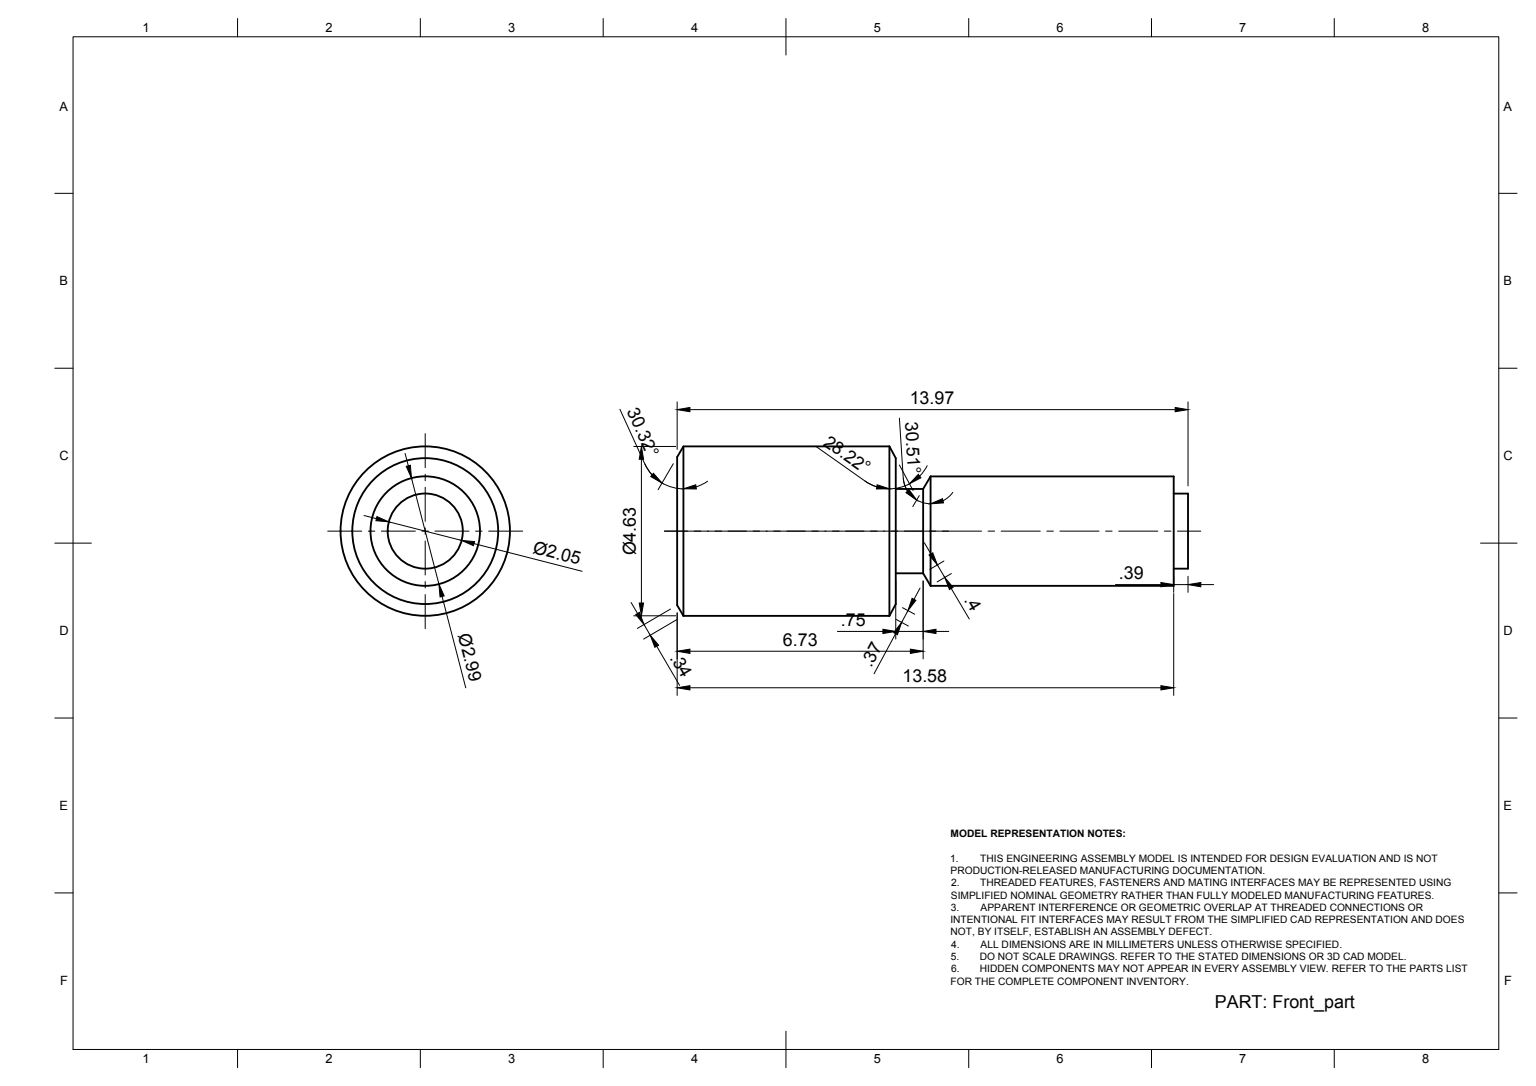
ISO-10303-21;
HEADER;
/* Generated by software containing ST-Developer
 * from STEP Tools, Inc. (www.steptools.com) 
 */

FILE_DESCRIPTION(
/* description */ (''),
/* implementation_level */ '2;1');

FILE_NAME(
/* name */ 'Front_part.step',
/* time_stamp */ '2026-10-05T00:51:14-07:00',
/* author */ (''),
/* organization */ (''),
/* preprocessor_version */ 'ST-DEVELOPER v20.2',
/* originating_system */ 'Autodesk Translation Framework v15.15.0.0',
/* authorisation */ '');

FILE_SCHEMA (('AUTOMOTIVE_DESIGN { 1 0 10303 214 3 1 1 }'));
ENDSEC;

DATA;
#10=MECHANICAL_DESIGN_GEOMETRIC_PRESENTATION_REPRESENTATION('',(#390),#4613);
#55=CONICAL_SURFACE('',#1766,1.32430878211522,1.03823317791294);
#56=CONICAL_SURFACE('',#1773,2.15547938178353,1.07831899445638);
#57=CONICAL_SURFACE('',#1777,2.17072351166958,1.04154954596305);
#77=FACE_BOUND('',#558,.T.);
#78=FACE_BOUND('',#563,.T.);
#79=FACE_BOUND('',#569,.T.);
#105=PLANE('',#1771);
#106=PLANE('',#1779);
#107=PLANE('',#1783);
#108=PLANE('',#1784);
#109=PLANE('',#1788);
#191=LINE('',#2638,#274);
#192=LINE('',#2643,#275);
#193=LINE('',#2650,#276);
#194=LINE('',#2654,#277);
#195=LINE('',#2657,#278);
#196=LINE('',#2665,#279);
#197=LINE('',#2673,#280);
#198=LINE('',#2678,#281);
#274=VECTOR('',#2082,1.32430878211522);
#275=VECTOR('',#2089,1.15283995859749);
#276=VECTOR('',#2098,2.15547938178353);
#277=VECTOR('',#2103,2.3164003912567);
#278=VECTOR('',#2106,2.17072351166958);
#279=VECTOR('',#2117,0.94209020647254);
#280=VECTOR('',#2128,1.02706997925809);
#281=VECTOR('',#2135,1.49577760563294);
#345=CYLINDRICAL_SURFACE('',#1769,1.15283995859749);
#346=CYLINDRICAL_SURFACE('',#1775,2.3164003912567);
#347=CYLINDRICAL_SURFACE('',#1781,0.94209020647254);
#348=CYLINDRICAL_SURFACE('',#1786,1.02706997925809);
#349=CYLINDRICAL_SURFACE('',#1790,1.49577760563294);
#374=SHAPE_REPRESENTATION_RELATIONSHIP('SRR','None',#4648,#382);
#382=ADVANCED_BREP_SHAPE_REPRESENTATION('',(#398),#4608);
#390=STYLED_ITEM('',(#4695),#398);
#398=MANIFOLD_SOLID_BREP('Body1',#1597);
#439=FACE_OUTER_BOUND('',#555,.T.);
#440=FACE_OUTER_BOUND('',#556,.T.);
#441=FACE_OUTER_BOUND('',#557,.T.);
#442=FACE_OUTER_BOUND('',#559,.T.);
#443=FACE_OUTER_BOUND('',#560,.T.);
#444=FACE_OUTER_BOUND('',#561,.T.);
#445=FACE_OUTER_BOUND('',#562,.T.);
#446=FACE_OUTER_BOUND('',#564,.T.);
#447=FACE_OUTER_BOUND('',#565,.T.);
#448=FACE_OUTER_BOUND('',#566,.T.);
#449=FACE_OUTER_BOUND('',#567,.T.);
#450=FACE_OUTER_BOUND('',#568,.T.);
#451=FACE_OUTER_BOUND('',#570,.T.);
#555=EDGE_LOOP('',(#1205,#1206,#1207,#1208));
#556=EDGE_LOOP('',(#1209,#1210,#1211,#1212));
#557=EDGE_LOOP('',(#1213));
#558=EDGE_LOOP('',(#1214));
#559=EDGE_LOOP('',(#1215,#1216,#1217,#1218));
#560=EDGE_LOOP('',(#1219,#1220,#1221,#1222));
#561=EDGE_LOOP('',(#1223,#1224,#1225,#1226));
#562=EDGE_LOOP('',(#1227));
#563=EDGE_LOOP('',(#1228));
#564=EDGE_LOOP('',(#1229,#1230,#1231,#1232));
#565=EDGE_LOOP('',(#1233));
#566=EDGE_LOOP('',(#1234));
#567=EDGE_LOOP('',(#1235,#1236,#1237,#1238));
#568=EDGE_LOOP('',(#1239));
#569=EDGE_LOOP('',(#1240));
#570=EDGE_LOOP('',(#1241,#1242,#1243,#1244));
#673=CIRCLE('',#1767,1.49577760563294);
#674=CIRCLE('',#1768,1.15283995859749);
#675=CIRCLE('',#1770,1.15283995859749);
#676=CIRCLE('',#1772,1.99455837231036);
#677=CIRCLE('',#1774,2.3164003912567);
#678=CIRCLE('',#1776,2.3164003912567);
#679=CIRCLE('',#1778,2.02504663208246);
#680=CIRCLE('',#1780,0.94209020647254);
#681=CIRCLE('',#1782,0.94209020647254);
#682=CIRCLE('',#1785,1.02706997925809);
#683=CIRCLE('',#1787,1.02706997925809);
#684=CIRCLE('',#1789,1.49577760563294);
#774=VERTEX_POINT('',#2635);
#775=VERTEX_POINT('',#2637);
#776=VERTEX_POINT('',#2641);
#777=VERTEX_POINT('',#2645);
#778=VERTEX_POINT('',#2648);
#779=VERTEX_POINT('',#2652);
#780=VERTEX_POINT('',#2656);
#781=VERTEX_POINT('',#2660);
#782=VERTEX_POINT('',#2663);
#783=VERTEX_POINT('',#2668);
#784=VERTEX_POINT('',#2671);
#785=VERTEX_POINT('',#2675);
#930=EDGE_CURVE('',#774,#774,#673,.T.);
#931=EDGE_CURVE('',#774,#775,#191,.T.);
#932=EDGE_CURVE('',#775,#775,#674,.T.);
#933=EDGE_CURVE('',#776,#776,#675,.T.);
#934=EDGE_CURVE('',#776,#775,#192,.T.);
#935=EDGE_CURVE('',#777,#777,#676,.T.);
#936=EDGE_CURVE('',#778,#778,#677,.T.);
#937=EDGE_CURVE('',#778,#777,#193,.T.);
#938=EDGE_CURVE('',#779,#779,#678,.T.);
#939=EDGE_CURVE('',#779,#778,#194,.T.);
#940=EDGE_CURVE('',#779,#780,#195,.T.);
#941=EDGE_CURVE('',#780,#780,#679,.T.);
#942=EDGE_CURVE('',#781,#781,#680,.T.);
#943=EDGE_CURVE('',#782,#782,#681,.T.);
#944=EDGE_CURVE('',#782,#781,#196,.T.);
#945=EDGE_CURVE('',#783,#783,#682,.T.);
#946=EDGE_CURVE('',#784,#784,#683,.T.);
#947=EDGE_CURVE('',#784,#783,#197,.T.);
#948=EDGE_CURVE('',#785,#785,#684,.T.);
#949=EDGE_CURVE('',#774,#785,#198,.T.);
#1205=ORIENTED_EDGE('',*,*,#930,.T.);
#1206=ORIENTED_EDGE('',*,*,#931,.T.);
#1207=ORIENTED_EDGE('',*,*,#932,.F.);
#1208=ORIENTED_EDGE('',*,*,#931,.F.);
#1209=ORIENTED_EDGE('',*,*,#933,.F.);
#1210=ORIENTED_EDGE('',*,*,#934,.T.);
#1211=ORIENTED_EDGE('',*,*,#932,.T.);
#1212=ORIENTED_EDGE('',*,*,#934,.F.);
#1213=ORIENTED_EDGE('',*,*,#935,.F.);
#1214=ORIENTED_EDGE('',*,*,#933,.T.);
#1215=ORIENTED_EDGE('',*,*,#936,.F.);
#1216=ORIENTED_EDGE('',*,*,#937,.T.);
#1217=ORIENTED_EDGE('',*,*,#935,.T.);
#1218=ORIENTED_EDGE('',*,*,#937,.F.);
#1219=ORIENTED_EDGE('',*,*,#938,.F.);
#1220=ORIENTED_EDGE('',*,*,#939,.T.);
#1221=ORIENTED_EDGE('',*,*,#936,.T.);
#1222=ORIENTED_EDGE('',*,*,#939,.F.);
#1223=ORIENTED_EDGE('',*,*,#938,.T.);
#1224=ORIENTED_EDGE('',*,*,#940,.T.);
#1225=ORIENTED_EDGE('',*,*,#941,.F.);
#1226=ORIENTED_EDGE('',*,*,#940,.F.);
#1227=ORIENTED_EDGE('',*,*,#941,.T.);
#1228=ORIENTED_EDGE('',*,*,#942,.F.);
#1229=ORIENTED_EDGE('',*,*,#943,.F.);
#1230=ORIENTED_EDGE('',*,*,#944,.T.);
#1231=ORIENTED_EDGE('',*,*,#942,.T.);
#1232=ORIENTED_EDGE('',*,*,#944,.F.);
#1233=ORIENTED_EDGE('',*,*,#943,.T.);
#1234=ORIENTED_EDGE('',*,*,#945,.F.);
#1235=ORIENTED_EDGE('',*,*,#946,.F.);
#1236=ORIENTED_EDGE('',*,*,#947,.T.);
#1237=ORIENTED_EDGE('',*,*,#945,.T.);
#1238=ORIENTED_EDGE('',*,*,#947,.F.);
#1239=ORIENTED_EDGE('',*,*,#948,.F.);
#1240=ORIENTED_EDGE('',*,*,#946,.T.);
#1241=ORIENTED_EDGE('',*,*,#930,.F.);
#1242=ORIENTED_EDGE('',*,*,#949,.T.);
#1243=ORIENTED_EDGE('',*,*,#948,.T.);
#1244=ORIENTED_EDGE('',*,*,#949,.F.);
#1524=ADVANCED_FACE('',(#439),#55,.T.);
#1525=ADVANCED_FACE('',(#440),#345,.T.);
#1526=ADVANCED_FACE('',(#441,#77),#105,.T.);
#1527=ADVANCED_FACE('',(#442),#56,.T.);
#1528=ADVANCED_FACE('',(#443),#346,.T.);
#1529=ADVANCED_FACE('',(#444),#57,.T.);
#1530=ADVANCED_FACE('',(#445,#78),#106,.T.);
#1531=ADVANCED_FACE('',(#446),#347,.F.);
#1532=ADVANCED_FACE('',(#447),#107,.T.);
#1533=ADVANCED_FACE('',(#448),#108,.T.);
#1534=ADVANCED_FACE('',(#449),#348,.T.);
#1535=ADVANCED_FACE('',(#450,#79),#109,.T.);
#1536=ADVANCED_FACE('',(#451),#349,.T.);
#1597=CLOSED_SHELL('',(#1524,#1525,#1526,#1527,#1528,#1529,#1530,#1531,
#1532,#1533,#1534,#1535,#1536));
#1765=AXIS2_PLACEMENT_3D('',#2633,#2076,#2077);
#1766=AXIS2_PLACEMENT_3D('',#2634,#2078,#2079);
#1767=AXIS2_PLACEMENT_3D('',#2636,#2080,#2081);
#1768=AXIS2_PLACEMENT_3D('',#2639,#2083,#2084);
#1769=AXIS2_PLACEMENT_3D('',#2640,#2085,#2086);
#1770=AXIS2_PLACEMENT_3D('',#2642,#2087,#2088);
#1771=AXIS2_PLACEMENT_3D('',#2644,#2090,#2091);
#1772=AXIS2_PLACEMENT_3D('',#2646,#2092,#2093);
#1773=AXIS2_PLACEMENT_3D('',#2647,#2094,#2095);
#1774=AXIS2_PLACEMENT_3D('',#2649,#2096,#2097);
#1775=AXIS2_PLACEMENT_3D('',#2651,#2099,#2100);
#1776=AXIS2_PLACEMENT_3D('',#2653,#2101,#2102);
#1777=AXIS2_PLACEMENT_3D('',#2655,#2104,#2105);
#1778=AXIS2_PLACEMENT_3D('',#2658,#2107,#2108);
#1779=AXIS2_PLACEMENT_3D('',#2659,#2109,#2110);
#1780=AXIS2_PLACEMENT_3D('',#2661,#2111,#2112);
#1781=AXIS2_PLACEMENT_3D('',#2662,#2113,#2114);
#1782=AXIS2_PLACEMENT_3D('',#2664,#2115,#2116);
#1783=AXIS2_PLACEMENT_3D('',#2666,#2118,#2119);
#1784=AXIS2_PLACEMENT_3D('',#2667,#2120,#2121);
#1785=AXIS2_PLACEMENT_3D('',#2669,#2122,#2123);
#1786=AXIS2_PLACEMENT_3D('',#2670,#2124,#2125);
#1787=AXIS2_PLACEMENT_3D('',#2672,#2126,#2127);
#1788=AXIS2_PLACEMENT_3D('',#2674,#2129,#2130);
#1789=AXIS2_PLACEMENT_3D('',#2676,#2131,#2132);
#1790=AXIS2_PLACEMENT_3D('',#2677,#2133,#2134);
#2076=DIRECTION('axis',(0.,0.,1.));
#2077=DIRECTION('refdir',(1.,0.,0.));
#2078=DIRECTION('center_axis',(-1.,0.,0.));
#2079=DIRECTION('ref_axis',(0.,0.,-1.));
#2080=DIRECTION('center_axis',(1.,0.,0.));
#2081=DIRECTION('ref_axis',(0.,0.,-1.));
#2082=DIRECTION('',(0.507743181153061,-1.05504360309624E-16,-0.861508480511115));
#2083=DIRECTION('center_axis',(1.,0.,0.));
#2084=DIRECTION('ref_axis',(0.,0.,-1.));
#2085=DIRECTION('center_axis',(1.,0.,0.));
#2086=DIRECTION('ref_axis',(0.,0.,-1.));
#2087=DIRECTION('center_axis',(1.,0.,0.));
#2088=DIRECTION('ref_axis',(0.,0.,-1.));
#2089=DIRECTION('',(-1.,0.,0.));
#2090=DIRECTION('center_axis',(-1.,0.,0.));
#2091=DIRECTION('ref_axis',(0.,0.,1.));
#2092=DIRECTION('center_axis',(1.,0.,0.));
#2093=DIRECTION('ref_axis',(0.,0.,-1.));
#2094=DIRECTION('center_axis',(1.,0.,0.));
#2095=DIRECTION('ref_axis',(0.,0.,-1.));
#2096=DIRECTION('center_axis',(1.,0.,0.));
#2097=DIRECTION('ref_axis',(0.,0.,-1.));
#2098=DIRECTION('',(-0.472810273503224,1.07911498508989E-16,-0.88116425555614));
#2099=DIRECTION('center_axis',(1.,0.,0.));
#2100=DIRECTION('ref_axis',(0.,0.,-1.));
#2101=DIRECTION('center_axis',(1.,0.,0.));
#2102=DIRECTION('ref_axis',(0.,0.,-1.));
#2103=DIRECTION('',(-1.,0.,0.));
#2104=DIRECTION('center_axis',(-1.,0.,0.));
#2105=DIRECTION('ref_axis',(0.,0.,-1.));
#2106=DIRECTION('',(0.504883315037955,-1.0570999352361E-16,-0.863187603129404));
#2107=DIRECTION('center_axis',(1.,0.,0.));
#2108=DIRECTION('ref_axis',(0.,0.,-1.));
#2109=DIRECTION('center_axis',(1.,0.,0.));
#2110=DIRECTION('ref_axis',(0.,0.,-1.));
#2111=DIRECTION('center_axis',(1.,0.,0.));
#2112=DIRECTION('ref_axis',(0.,0.,-1.));
#2113=DIRECTION('center_axis',(1.,0.,0.));
#2114=DIRECTION('ref_axis',(0.,0.,-1.));
#2115=DIRECTION('center_axis',(1.,0.,0.));
#2116=DIRECTION('ref_axis',(0.,0.,-1.));
#2117=DIRECTION('',(1.,0.,0.));
#2118=DIRECTION('center_axis',(1.,0.,0.));
#2119=DIRECTION('ref_axis',(0.,0.,-1.));
#2120=DIRECTION('center_axis',(-1.,0.,0.));
#2121=DIRECTION('ref_axis',(0.,0.,1.));
#2122=DIRECTION('center_axis',(1.,0.,0.));
#2123=DIRECTION('ref_axis',(0.,0.,-1.));
#2124=DIRECTION('center_axis',(1.,0.,0.));
#2125=DIRECTION('ref_axis',(0.,0.,-1.));
#2126=DIRECTION('center_axis',(1.,0.,0.));
#2127=DIRECTION('ref_axis',(0.,0.,-1.));
#2128=DIRECTION('',(-1.,0.,0.));
#2129=DIRECTION('center_axis',(-1.,0.,0.));
#2130=DIRECTION('ref_axis',(0.,0.,1.));
#2131=DIRECTION('center_axis',(1.,0.,0.));
#2132=DIRECTION('ref_axis',(0.,0.,-1.));
#2133=DIRECTION('center_axis',(1.,0.,0.));
#2134=DIRECTION('ref_axis',(0.,0.,-1.));
#2135=DIRECTION('',(-1.,0.,0.));
#2633=CARTESIAN_POINT('',(0.,0.,0.));
#2634=CARTESIAN_POINT('Origin',(-9.8399217662475,0.,0.));
#2635=CARTESIAN_POINT('',(-9.94097953629964,-1.83179925697468E-16,1.49577760563294));
#2636=CARTESIAN_POINT('Origin',(-9.94097953629964,0.,0.));
#2637=CARTESIAN_POINT('',(-9.73886399619536,-1.41182176522558E-16,1.15283995859749));
#2638=CARTESIAN_POINT('',(-9.8399217662475,1.62181051110013E-16,1.32430878211522));
#2639=CARTESIAN_POINT('Origin',(-9.73886399619536,0.,0.));
#2640=CARTESIAN_POINT('Origin',(-9.36350656457311,0.,0.));
#2641=CARTESIAN_POINT('',(-8.98814913295086,-1.41182176522558E-16,1.15283995859749));
#2642=CARTESIAN_POINT('Origin',(-8.98814913295086,0.,0.));
#2643=CARTESIAN_POINT('',(-9.36350656457311,-1.41182176522558E-16,1.15283995859749));
#2644=CARTESIAN_POINT('Origin',(-8.98814913295086,0.,-1.99455837231036));
#2645=CARTESIAN_POINT('',(-8.98814913295086,-2.44262952636244E-16,1.99455837231036));
#2646=CARTESIAN_POINT('Origin',(-8.98814913295086,0.,0.));
#2647=CARTESIAN_POINT('Origin',(-8.90180302208485,0.,0.));
#2648=CARTESIAN_POINT('',(-8.81545691121883,-2.83677232469619E-16,2.3164003912567));
#2649=CARTESIAN_POINT('Origin',(-8.81545691121883,0.,0.));
#2650=CARTESIAN_POINT('',(-8.90180302208485,-2.63970092552932E-16,2.15547938178353));
#2651=CARTESIAN_POINT('Origin',(-5.99766844795496,0.,0.));
#2652=CARTESIAN_POINT('',(-3.17987998469109,-2.83677232469619E-16,2.3164003912567));
#2653=CARTESIAN_POINT('Origin',(-3.17987998469109,0.,0.));
#2654=CARTESIAN_POINT('',(-5.99766844795496,-2.83677232469619E-16,2.3164003912567));
#2655=CARTESIAN_POINT('Origin',(-3.09467275323448,0.,0.));
#2656=CARTESIAN_POINT('',(-3.00946552177786,-2.47996687610391E-16,2.02504663208246));
#2657=CARTESIAN_POINT('',(-3.09467275323448,2.65836960040005E-16,2.17072351166958));
#2658=CARTESIAN_POINT('Origin',(-3.00946552177786,0.,0.));
#2659=CARTESIAN_POINT('Origin',(-3.00946552177786,0.,-0.94209020647254));
#2660=CARTESIAN_POINT('',(-3.00946552177786,-1.15372775586467E-16,0.94209020647254));
#2661=CARTESIAN_POINT('Origin',(-3.00946552177786,0.,0.));
#2662=CARTESIAN_POINT('Origin',(-3.89726990114842,0.,0.));
#2663=CARTESIAN_POINT('',(-4.78507428051899,-1.15372775586467E-16,0.94209020647254));
#2664=CARTESIAN_POINT('Origin',(-4.78507428051899,0.,0.));
#2665=CARTESIAN_POINT('',(-3.89726990114842,-1.15372775586467E-16,0.94209020647254));
#2666=CARTESIAN_POINT('Origin',(-4.78507428051899,0.,0.));
#2667=CARTESIAN_POINT('Origin',(-16.9835276458929,0.,-1.02706997925809));
#2668=CARTESIAN_POINT('',(-16.9835276458929,-1.25779796259876E-16,1.02706997925809));
#2669=CARTESIAN_POINT('Origin',(-16.9835276458929,0.,0.));
#2670=CARTESIAN_POINT('Origin',(-16.7880966836618,0.,0.));
#2671=CARTESIAN_POINT('',(-16.5926657214308,-1.25779796259876E-16,1.02706997925809));
#2672=CARTESIAN_POINT('Origin',(-16.5926657214308,0.,0.));
#2673=CARTESIAN_POINT('',(-16.7880966836618,-1.25779796259876E-16,1.02706997925809));
#2674=CARTESIAN_POINT('Origin',(-16.5926657214308,0.,-1.49577760563294));
#2675=CARTESIAN_POINT('',(-16.5926657214308,-1.83179925697468E-16,1.49577760563294));
#2676=CARTESIAN_POINT('Origin',(-16.5926657214308,0.,0.));
#2677=CARTESIAN_POINT('Origin',(-13.2668226288652,0.,0.));
#2678=CARTESIAN_POINT('',(-13.2668226288652,-1.83179925697467E-16,1.49577760563294));
#4598=UNCERTAINTY_MEASURE_WITH_UNIT(LENGTH_MEASURE(0.01),#4614,
'DISTANCE_ACCURACY_VALUE',
'Maximum model space distance between geometric entities at asserted c
onnectivities');
#4603=UNCERTAINTY_MEASURE_WITH_UNIT(LENGTH_MEASURE(0.01),#4614,
'DISTANCE_ACCURACY_VALUE',
'Maximum model space distance between geometric entities at asserted c
onnectivities');
#4608=(
GEOMETRIC_REPRESENTATION_CONTEXT(3)
GLOBAL_UNCERTAINTY_ASSIGNED_CONTEXT((#4598))
GLOBAL_UNIT_ASSIGNED_CONTEXT((#4614,#4616,#4617))
REPRESENTATION_CONTEXT('','3D')
);
#4613=(
GEOMETRIC_REPRESENTATION_CONTEXT(3)
GLOBAL_UNCERTAINTY_ASSIGNED_CONTEXT((#4603))
GLOBAL_UNIT_ASSIGNED_CONTEXT((#4614,#4616,#4617))
REPRESENTATION_CONTEXT('','3D')
);
#4614=(
LENGTH_UNIT()
NAMED_UNIT(*)
SI_UNIT(.MILLI.,.METRE.)
);
#4616=(
NAMED_UNIT(*)
PLANE_ANGLE_UNIT()
SI_UNIT($,.RADIAN.)
);
#4617=(
NAMED_UNIT(*)
SI_UNIT($,.STERADIAN.)
SOLID_ANGLE_UNIT()
);
#4622=SHAPE_DEFINITION_REPRESENTATION(#4631,#4648);
#4631=PRODUCT_DEFINITION_SHAPE('',$,#4658);
#4648=SHAPE_REPRESENTATION('',(#1765),#4608);
#4653=PRODUCT_DEFINITION_CONTEXT('part definition',#4682,'design');
#4658=PRODUCT_DEFINITION('Front_part','Front_part',#4667,#4653);
#4667=PRODUCT_DEFINITION_FORMATION('',$,#4688);
#4682=APPLICATION_CONTEXT(
'Core Data for Automotive Mechanical Design Process');
#4683=PRODUCT_CONTEXT('part definition',#4682,'mechanical');
#4688=PRODUCT('Front_part','Front_part',$,(#4683));
#4695=PRESENTATION_STYLE_ASSIGNMENT((#4700));
#4700=SURFACE_STYLE_USAGE(.BOTH.,#4705);
#4705=SURFACE_SIDE_STYLE('',(#4710));
#4710=SURFACE_STYLE_FILL_AREA(#4715);
#4715=FILL_AREA_STYLE('Opaque(255,255,255)',(#4720));
#4720=FILL_AREA_STYLE_COLOUR('Opaque(255,255,255)',#4725);
#4725=COLOUR_RGB('Opaque(255,255,255)', 0.66274510, 0.83137255, 0.94901961);
ENDSEC;
END-ISO-10303-21;
